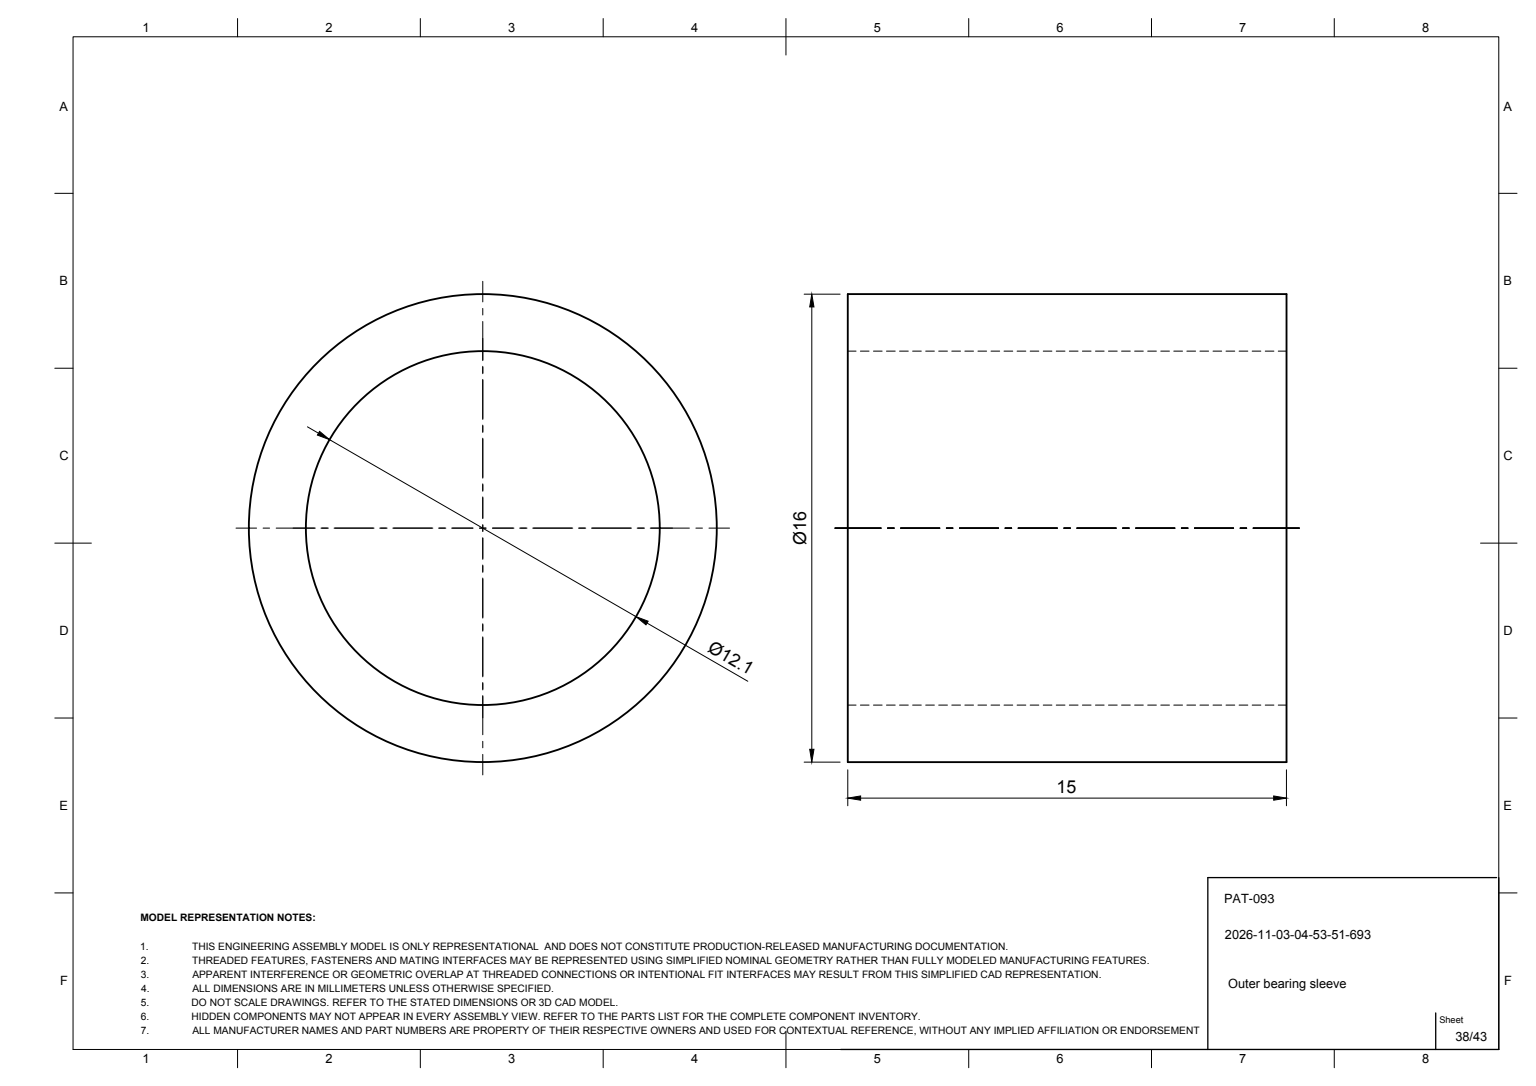
ISO-10303-21;
HEADER;
/* Generated by software containing ST-Developer
 * from STEP Tools, Inc. (www.steptools.com) 
 */

FILE_DESCRIPTION(
/* description */ ('Self-centering screw clamp'),
/* implementation_level */ '2;1');

FILE_NAME(
/* name */ 'Outer bearing sleeve.step',
/* time_stamp */ '2026-10-28T03:25:31-07:00',
/* author */ (''),
/* organization */ (''),
/* preprocessor_version */ 'ST-DEVELOPER v20.2',
/* originating_system */ 'Autodesk Translation Framework v15.17.0.0',
/* authorisation */ '');

FILE_SCHEMA (('AUTOMOTIVE_DESIGN { 1 0 10303 214 3 1 1 }'));
ENDSEC;

DATA;
#10=MECHANICAL_DESIGN_GEOMETRIC_PRESENTATION_REPRESENTATION('',(#664),#16799);
#575=SHAPE_REPRESENTATION_RELATIONSHIP('SRR','None',#17053,#616);
#616=ADVANCED_BREP_SHAPE_REPRESENTATION('',(#711),#16791);
#664=STYLED_ITEM('',(#17326),#711);
#711=MANIFOLD_SOLID_BREP('Body1',#9116);
#999=FACE_BOUND('',#2504,.T.);
#1000=FACE_BOUND('',#2506,.T.);
#1236=PLANE('',#10542);
#1237=PLANE('',#10543);
#1716=FACE_OUTER_BOUND('',#2501,.T.);
#1717=FACE_OUTER_BOUND('',#2502,.T.);
#1718=FACE_OUTER_BOUND('',#2503,.T.);
#1719=FACE_OUTER_BOUND('',#2505,.T.);
#2501=EDGE_LOOP('',(#8109,#8110,#8111,#8112));
#2502=EDGE_LOOP('',(#8113,#8114,#8115,#8116));
#2503=EDGE_LOOP('',(#8117));
#2504=EDGE_LOOP('',(#8118));
#2505=EDGE_LOOP('',(#8119));
#2506=EDGE_LOOP('',(#8120));
#3082=LINE('',#16210,#3655);
#3083=LINE('',#16216,#3656);
#3655=VECTOR('',#13179,0.605);
#3656=VECTOR('',#13186,0.8);
#4191=CIRCLE('',#10537,0.605);
#4192=CIRCLE('',#10538,0.605);
#4193=CIRCLE('',#10540,0.8);
#4194=CIRCLE('',#10541,0.8);
#4896=VERTEX_POINT('',#16207);
#4897=VERTEX_POINT('',#16209);
#4898=VERTEX_POINT('',#16213);
#4899=VERTEX_POINT('',#16215);
#5979=EDGE_CURVE('',#4896,#4896,#4191,.T.);
#5980=EDGE_CURVE('',#4896,#4897,#3082,.T.);
#5981=EDGE_CURVE('',#4897,#4897,#4192,.T.);
#5982=EDGE_CURVE('',#4898,#4898,#4193,.T.);
#5983=EDGE_CURVE('',#4898,#4899,#3083,.T.);
#5984=EDGE_CURVE('',#4899,#4899,#4194,.T.);
#8109=ORIENTED_EDGE('',*,*,#5979,.F.);
#8110=ORIENTED_EDGE('',*,*,#5980,.T.);
#8111=ORIENTED_EDGE('',*,*,#5981,.T.);
#8112=ORIENTED_EDGE('',*,*,#5980,.F.);
#8113=ORIENTED_EDGE('',*,*,#5982,.F.);
#8114=ORIENTED_EDGE('',*,*,#5983,.T.);
#8115=ORIENTED_EDGE('',*,*,#5984,.T.);
#8116=ORIENTED_EDGE('',*,*,#5983,.F.);
#8117=ORIENTED_EDGE('',*,*,#5982,.T.);
#8118=ORIENTED_EDGE('',*,*,#5979,.T.);
#8119=ORIENTED_EDGE('',*,*,#5984,.F.);
#8120=ORIENTED_EDGE('',*,*,#5981,.F.);
#8553=CYLINDRICAL_SURFACE('',#10536,0.605);
#8554=CYLINDRICAL_SURFACE('',#10539,0.8);
#9014=ADVANCED_FACE('',(#1716),#8553,.F.);
#9015=ADVANCED_FACE('',(#1717),#8554,.T.);
#9016=ADVANCED_FACE('',(#1718,#999),#1236,.T.);
#9017=ADVANCED_FACE('',(#1719,#1000),#1237,.F.);
#9116=CLOSED_SHELL('',(#9014,#9015,#9016,#9017));
#10535=AXIS2_PLACEMENT_3D('',#16205,#13173,#13174);
#10536=AXIS2_PLACEMENT_3D('',#16206,#13175,#13176);
#10537=AXIS2_PLACEMENT_3D('',#16208,#13177,#13178);
#10538=AXIS2_PLACEMENT_3D('',#16211,#13180,#13181);
#10539=AXIS2_PLACEMENT_3D('',#16212,#13182,#13183);
#10540=AXIS2_PLACEMENT_3D('',#16214,#13184,#13185);
#10541=AXIS2_PLACEMENT_3D('',#16217,#13187,#13188);
#10542=AXIS2_PLACEMENT_3D('',#16218,#13189,#13190);
#10543=AXIS2_PLACEMENT_3D('',#16219,#13191,#13192);
#13173=DIRECTION('axis',(0.,0.,1.));
#13174=DIRECTION('refdir',(1.,0.,0.));
#13175=DIRECTION('center_axis',(1.,0.,0.));
#13176=DIRECTION('ref_axis',(0.,0.,-1.));
#13177=DIRECTION('center_axis',(-1.,0.,0.));
#13178=DIRECTION('ref_axis',(0.,0.,-1.));
#13179=DIRECTION('',(-1.,0.,0.));
#13180=DIRECTION('center_axis',(-1.,0.,0.));
#13181=DIRECTION('ref_axis',(0.,0.,-1.));
#13182=DIRECTION('center_axis',(1.,0.,0.));
#13183=DIRECTION('ref_axis',(0.,0.,-1.));
#13184=DIRECTION('center_axis',(1.,0.,0.));
#13185=DIRECTION('ref_axis',(0.,0.,-1.));
#13186=DIRECTION('',(-1.,0.,0.));
#13187=DIRECTION('center_axis',(1.,0.,0.));
#13188=DIRECTION('ref_axis',(0.,0.,-1.));
#13189=DIRECTION('center_axis',(1.,0.,0.));
#13190=DIRECTION('ref_axis',(0.,0.,-1.));
#13191=DIRECTION('center_axis',(1.,0.,0.));
#13192=DIRECTION('ref_axis',(0.,0.,-1.));
#16205=CARTESIAN_POINT('',(0.,0.,0.));
#16206=CARTESIAN_POINT('Origin',(-13.5,0.,4.));
#16207=CARTESIAN_POINT('',(-12.,-7.40911313484149E-17,4.605));
#16208=CARTESIAN_POINT('Origin',(-12.,0.,4.));
#16209=CARTESIAN_POINT('',(-13.5,-7.40911313484149E-17,4.605));
#16210=CARTESIAN_POINT('',(-13.5,-7.40911313484149E-17,4.605));
#16211=CARTESIAN_POINT('Origin',(-13.5,0.,4.));
#16212=CARTESIAN_POINT('Origin',(-13.5,0.,4.));
#16213=CARTESIAN_POINT('',(-12.,-9.79717439317882E-17,4.8));
#16214=CARTESIAN_POINT('Origin',(-12.,0.,4.));
#16215=CARTESIAN_POINT('',(-13.5,-9.79717439317882E-17,4.8));
#16216=CARTESIAN_POINT('',(-13.5,-9.79717439317882E-17,4.8));
#16217=CARTESIAN_POINT('Origin',(-13.5,0.,4.));
#16218=CARTESIAN_POINT('Origin',(-12.,0.,4.));
#16219=CARTESIAN_POINT('Origin',(-13.5,0.,4.));
#16742=UNCERTAINTY_MEASURE_WITH_UNIT(LENGTH_MEASURE(0.001),#16800,
'DISTANCE_ACCURACY_VALUE',
'Maximum model space distance between geometric entities at asserted c
onnectivities');
#16750=UNCERTAINTY_MEASURE_WITH_UNIT(LENGTH_MEASURE(0.001),#16800,
'DISTANCE_ACCURACY_VALUE',
'Maximum model space distance between geometric entities at asserted c
onnectivities');
#16791=(
GEOMETRIC_REPRESENTATION_CONTEXT(3)
GLOBAL_UNCERTAINTY_ASSIGNED_CONTEXT((#16742))
GLOBAL_UNIT_ASSIGNED_CONTEXT((#16800,#16802,#16803))
REPRESENTATION_CONTEXT('','3D')
);
#16799=(
GEOMETRIC_REPRESENTATION_CONTEXT(3)
GLOBAL_UNCERTAINTY_ASSIGNED_CONTEXT((#16750))
GLOBAL_UNIT_ASSIGNED_CONTEXT((#16800,#16802,#16803))
REPRESENTATION_CONTEXT('','3D')
);
#16800=(
LENGTH_UNIT()
NAMED_UNIT(*)
SI_UNIT(.CENTI.,.METRE.)
);
#16802=(
NAMED_UNIT(*)
PLANE_ANGLE_UNIT()
SI_UNIT($,.RADIAN.)
);
#16803=(
NAMED_UNIT(*)
SI_UNIT($,.STERADIAN.)
SOLID_ANGLE_UNIT()
);
#16844=SHAPE_DEFINITION_REPRESENTATION(#16899,#17053);
#16899=PRODUCT_DEFINITION_SHAPE('',$,#17102);
#17053=SHAPE_REPRESENTATION('',(#10535),#16791);
#17061=PRODUCT_DEFINITION_CONTEXT('part definition',#17207,'design');
#17102=PRODUCT_DEFINITION('Outer bearing sleeve','Outer bearing sleeve',
#17150,#17061);
#17150=PRODUCT_DEFINITION_FORMATION('',$,#17249);
#17207=APPLICATION_CONTEXT(
'Core Data for Automotive Mechanical Design Process');
#17208=PRODUCT_CONTEXT('part definition',#17207,'mechanical');
#17249=PRODUCT('Outer bearing sleeve','Outer bearing sleeve',
'Outer bearing sleeve',(#17208));
#17320=COLOUR_RGB('Grey',0.48,0.52,0.57);
#17321=FILL_AREA_STYLE_COLOUR('',#17320);
#17322=FILL_AREA_STYLE('',(#17321));
#17323=SURFACE_STYLE_FILL_AREA(#17322);
#17324=SURFACE_SIDE_STYLE('',(#17323));
#17325=SURFACE_STYLE_USAGE(.BOTH.,#17324);
#17326=PRESENTATION_STYLE_ASSIGNMENT((#17325));
ENDSEC;
END-ISO-10303-21;
